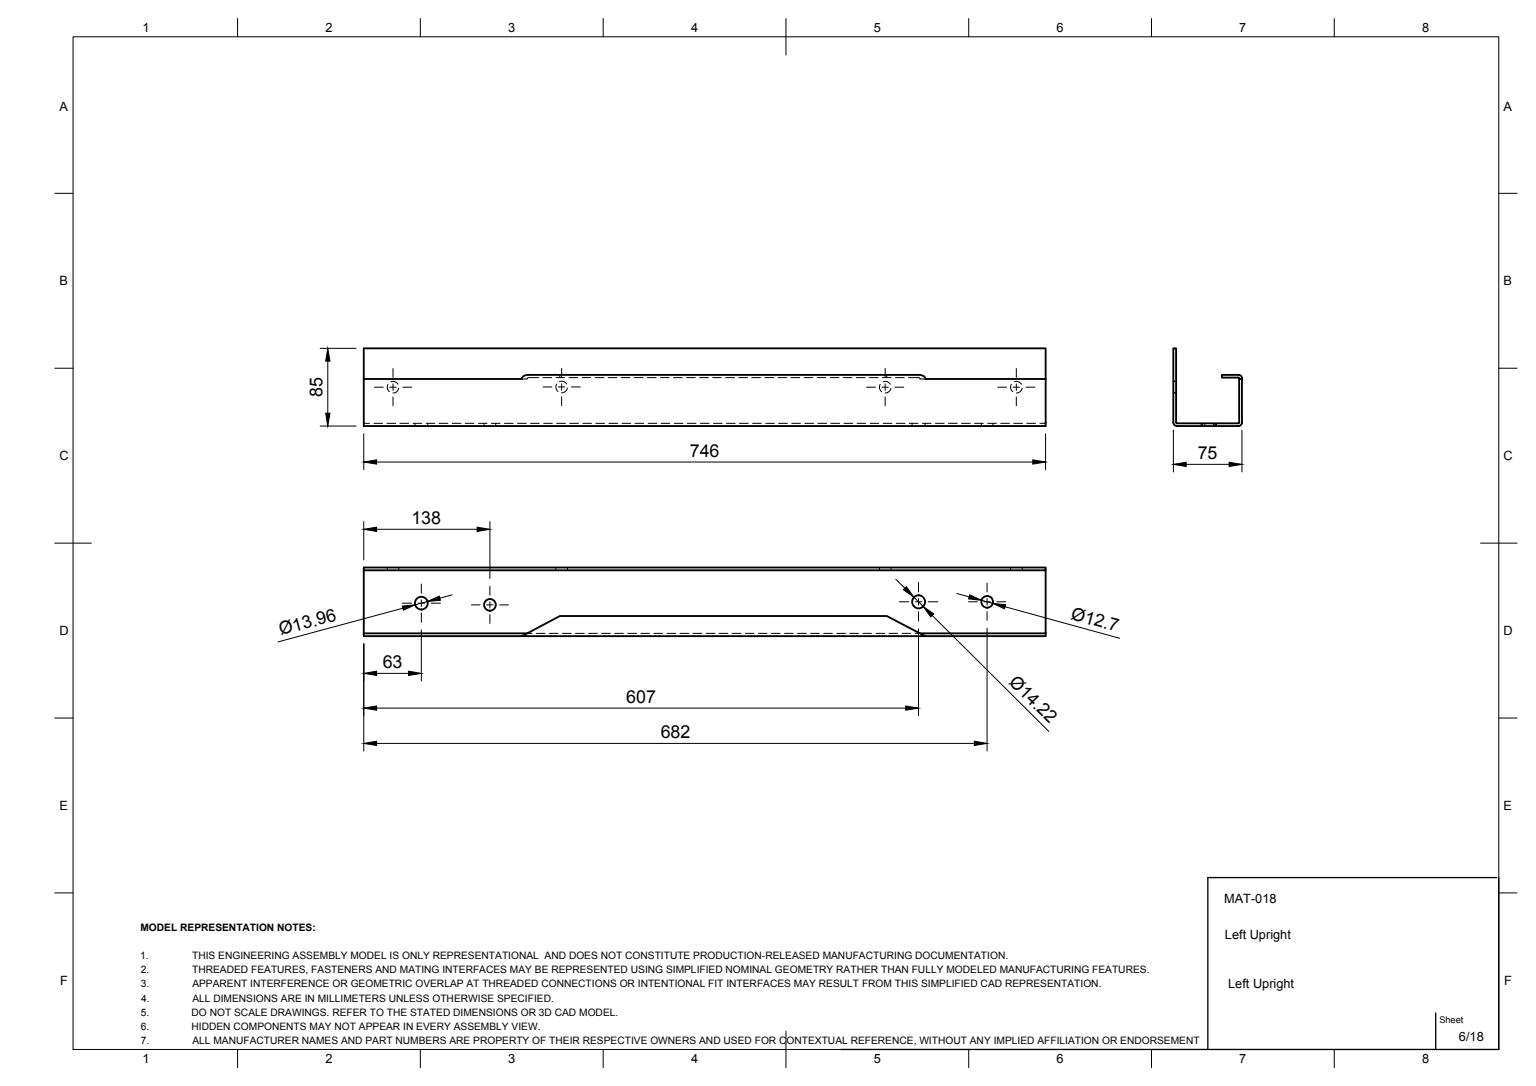
ISO-10303-21;
HEADER;
/* Generated by software containing ST-Developer
 * from STEP Tools, Inc. (www.steptools.com) 
 */

FILE_DESCRIPTION(
/* description */ ('STEP AP214'),
/* implementation_level */ '2;1');

FILE_NAME(
/* name */ 'Left Upright.step',
/* time_stamp */ '2026-11-14T06:16:09-08:00',
/* author */ (''),
/* organization */ (''),
/* preprocessor_version */ 'ST-DEVELOPER v20.2',
/* originating_system */ 'Autodesk Translation Framework v15.17.0.0',
/* authorisation */ '');

FILE_SCHEMA (('AUTOMOTIVE_DESIGN { 1 0 10303 214 3 1 1 }'));
ENDSEC;

DATA;
#10=MECHANICAL_DESIGN_GEOMETRIC_PRESENTATION_REPRESENTATION('',(#350),#18006);
#272=ELLIPSE('',#10126,8.64513309637285,4.00000000000059);
#273=ELLIPSE('',#10127,8.53586336233429,3.99999999999978);
#274=ELLIPSE('',#10140,2.1339658405822,0.999999999999361);
#275=ELLIPSE('',#10141,2.16128327409315,1.00000000000008);
#318=SHAPE_REPRESENTATION_RELATIONSHIP('SRR','None',#18074,#334);
#334=ADVANCED_BREP_SHAPE_REPRESENTATION('',(#366),#17991);
#350=STYLED_ITEM('',(#18171),#366);
#366=MANIFOLD_SOLID_BREP('Body1',#9559);
#433=FACE_BOUND('',#1692,.T.);
#434=FACE_BOUND('',#1693,.T.);
#435=FACE_BOUND('',#1694,.T.);
#436=FACE_BOUND('',#1695,.T.);
#437=FACE_BOUND('',#1698,.T.);
#438=FACE_BOUND('',#1699,.T.);
#439=FACE_BOUND('',#1700,.T.);
#440=FACE_BOUND('',#1701,.T.);
#441=FACE_BOUND('',#1704,.T.);
#442=FACE_BOUND('',#1705,.T.);
#443=FACE_BOUND('',#1706,.T.);
#444=FACE_BOUND('',#1707,.T.);
#445=FACE_BOUND('',#1710,.T.);
#446=FACE_BOUND('',#1711,.T.);
#447=FACE_BOUND('',#1712,.T.);
#448=FACE_BOUND('',#1713,.T.);
#638=PLANE('',#10105);
#639=PLANE('',#10106);
#640=PLANE('',#10109);
#641=PLANE('',#10110);
#642=PLANE('',#10113);
#643=PLANE('',#10114);
#644=PLANE('',#10117);
#645=PLANE('',#10118);
#646=PLANE('',#10121);
#647=PLANE('',#10122);
#648=PLANE('',#10123);
#649=PLANE('',#10124);
#650=PLANE('',#10128);
#651=PLANE('',#10130);
#652=PLANE('',#10132);
#653=PLANE('',#10133);
#654=PLANE('',#10134);
#655=PLANE('',#10136);
#656=PLANE('',#10138);
#657=PLANE('',#10142);
#658=PLANE('',#10143);
#659=PLANE('',#10144);
#660=PLANE('',#10145);
#661=PLANE('',#10146);
#1038=FACE_OUTER_BOUND('',#1668,.T.);
#1039=FACE_OUTER_BOUND('',#1669,.T.);
#1040=FACE_OUTER_BOUND('',#1670,.T.);
#1041=FACE_OUTER_BOUND('',#1671,.T.);
#1042=FACE_OUTER_BOUND('',#1672,.T.);
#1043=FACE_OUTER_BOUND('',#1673,.T.);
#1044=FACE_OUTER_BOUND('',#1674,.T.);
#1045=FACE_OUTER_BOUND('',#1675,.T.);
#1046=FACE_OUTER_BOUND('',#1676,.T.);
#1047=FACE_OUTER_BOUND('',#1677,.T.);
#1048=FACE_OUTER_BOUND('',#1678,.T.);
#1049=FACE_OUTER_BOUND('',#1679,.T.);
#1050=FACE_OUTER_BOUND('',#1680,.T.);
#1051=FACE_OUTER_BOUND('',#1681,.T.);
#1052=FACE_OUTER_BOUND('',#1682,.T.);
#1053=FACE_OUTER_BOUND('',#1683,.T.);
#1054=FACE_OUTER_BOUND('',#1684,.T.);
#1055=FACE_OUTER_BOUND('',#1685,.T.);
#1056=FACE_OUTER_BOUND('',#1686,.T.);
#1057=FACE_OUTER_BOUND('',#1687,.T.);
#1058=FACE_OUTER_BOUND('',#1688,.T.);
#1059=FACE_OUTER_BOUND('',#1689,.T.);
#1060=FACE_OUTER_BOUND('',#1690,.T.);
#1061=FACE_OUTER_BOUND('',#1691,.T.);
#1062=FACE_OUTER_BOUND('',#1696,.T.);
#1063=FACE_OUTER_BOUND('',#1697,.T.);
#1064=FACE_OUTER_BOUND('',#1702,.T.);
#1065=FACE_OUTER_BOUND('',#1703,.T.);
#1066=FACE_OUTER_BOUND('',#1708,.T.);
#1067=FACE_OUTER_BOUND('',#1709,.T.);
#1068=FACE_OUTER_BOUND('',#1714,.T.);
#1069=FACE_OUTER_BOUND('',#1715,.T.);
#1070=FACE_OUTER_BOUND('',#1716,.T.);
#1071=FACE_OUTER_BOUND('',#1717,.T.);
#1072=FACE_OUTER_BOUND('',#1718,.T.);
#1073=FACE_OUTER_BOUND('',#1719,.T.);
#1074=FACE_OUTER_BOUND('',#1720,.T.);
#1075=FACE_OUTER_BOUND('',#1721,.T.);
#1668=EDGE_LOOP('',(#7058,#7059,#7060,#7061));
#1669=EDGE_LOOP('',(#7062,#7063,#7064,#7065));
#1670=EDGE_LOOP('',(#7066,#7067,#7068,#7069));
#1671=EDGE_LOOP('',(#7070,#7071,#7072,#7073));
#1672=EDGE_LOOP('',(#7074,#7075,#7076,#7077));
#1673=EDGE_LOOP('',(#7078,#7079,#7080,#7081));
#1674=EDGE_LOOP('',(#7082,#7083,#7084,#7085));
#1675=EDGE_LOOP('',(#7086,#7087,#7088,#7089));
#1676=EDGE_LOOP('',(#7090,#7091,#7092,#7093));
#1677=EDGE_LOOP('',(#7094,#7095,#7096,#7097));
#1678=EDGE_LOOP('',(#7098,#7099,#7100,#7101));
#1679=EDGE_LOOP('',(#7102,#7103,#7104,#7105));
#1680=EDGE_LOOP('',(#7106,#7107,#7108,#7109));
#1681=EDGE_LOOP('',(#7110,#7111,#7112,#7113));
#1682=EDGE_LOOP('',(#7114,#7115,#7116,#7117));
#1683=EDGE_LOOP('',(#7118,#7119,#7120,#7121));
#1684=EDGE_LOOP('',(#7122,#7123,#7124,#7125));
#1685=EDGE_LOOP('',(#7126,#7127,#7128,#7129));
#1686=EDGE_LOOP('',(#7130,#7131,#7132,#7133));
#1687=EDGE_LOOP('',(#7134,#7135,#7136,#7137));
#1688=EDGE_LOOP('',(#7138,#7139,#7140,#7141));
#1689=EDGE_LOOP('',(#7142,#7143,#7144,#7145,#7146,#7147,#7148,#7149));
#1690=EDGE_LOOP('',(#7150,#7151,#7152,#7153));
#1691=EDGE_LOOP('',(#7154,#7155,#7156,#7157));
#1692=EDGE_LOOP('',(#7158));
#1693=EDGE_LOOP('',(#7159));
#1694=EDGE_LOOP('',(#7160));
#1695=EDGE_LOOP('',(#7161));
#1696=EDGE_LOOP('',(#7162,#7163,#7164,#7165));
#1697=EDGE_LOOP('',(#7166,#7167,#7168,#7169));
#1698=EDGE_LOOP('',(#7170));
#1699=EDGE_LOOP('',(#7171));
#1700=EDGE_LOOP('',(#7172));
#1701=EDGE_LOOP('',(#7173));
#1702=EDGE_LOOP('',(#7174,#7175,#7176,#7177));
#1703=EDGE_LOOP('',(#7178,#7179,#7180,#7181));
#1704=EDGE_LOOP('',(#7182));
#1705=EDGE_LOOP('',(#7183));
#1706=EDGE_LOOP('',(#7184));
#1707=EDGE_LOOP('',(#7185));
#1708=EDGE_LOOP('',(#7186,#7187,#7188,#7189));
#1709=EDGE_LOOP('',(#7190,#7191,#7192,#7193));
#1710=EDGE_LOOP('',(#7194));
#1711=EDGE_LOOP('',(#7195));
#1712=EDGE_LOOP('',(#7196));
#1713=EDGE_LOOP('',(#7197));
#1714=EDGE_LOOP('',(#7198,#7199,#7200,#7201));
#1715=EDGE_LOOP('',(#7202,#7203,#7204,#7205,#7206,#7207,#7208,#7209));
#1716=EDGE_LOOP('',(#7210,#7211,#7212,#7213));
#1717=EDGE_LOOP('',(#7214,#7215,#7216,#7217));
#1718=EDGE_LOOP('',(#7218,#7219,#7220,#7221));
#1719=EDGE_LOOP('',(#7222,#7223,#7224,#7225,#7226,#7227,#7228,#7229));
#1720=EDGE_LOOP('',(#7230,#7231,#7232,#7233,#7234,#7235,#7236,#7237));
#1721=EDGE_LOOP('',(#7238,#7239,#7240,#7241));
#2439=LINE('',#14730,#3163);
#2440=LINE('',#14736,#3164);
#2441=LINE('',#14742,#3165);
#2442=LINE('',#14748,#3166);
#2443=LINE('',#14754,#3167);
#2444=LINE('',#14760,#3168);
#2445=LINE('',#14766,#3169);
#2446=LINE('',#14772,#3170);
#2447=LINE('',#14777,#3171);
#2448=LINE('',#14779,#3172);
#2449=LINE('',#14781,#3173);
#2450=LINE('',#14782,#3174);
#2451=LINE('',#14786,#3175);
#2452=LINE('',#14790,#3176);
#2453=LINE('',#14794,#3177);
#2454=LINE('',#14796,#3178);
#2455=LINE('',#14797,#3179);
#2456=LINE('',#14801,#3180);
#2457=LINE('',#14805,#3181);
#2458=LINE('',#14809,#3182);
#2459=LINE('',#14811,#3183);
#2460=LINE('',#14812,#3184);
#2461=LINE('',#14816,#3185);
#2462=LINE('',#14820,#3186);
#2463=LINE('',#14823,#3187);
#2464=LINE('',#14824,#3188);
#2465=LINE('',#14831,#3189);
#2466=LINE('',#14832,#3190);
#2467=LINE('',#14833,#3191);
#2468=LINE('',#14837,#3192);
#2469=LINE('',#14839,#3193);
#2470=LINE('',#14841,#3194);
#2471=LINE('',#14842,#3195);
#2472=LINE('',#14845,#3196);
#2473=LINE('',#14847,#3197);
#2474=LINE('',#14848,#3198);
#2475=LINE('',#14851,#3199);
#2476=LINE('',#14853,#3200);
#2477=LINE('',#14854,#3201);
#2478=LINE('',#14860,#3202);
#2479=LINE('',#14863,#3203);
#2480=LINE('',#14865,#3204);
#2481=LINE('',#14866,#3205);
#2482=LINE('',#14867,#3206);
#2483=LINE('',#14868,#3207);
#2484=LINE('',#14870,#3208);
#2485=LINE('',#14872,#3209);
#2486=LINE('',#14874,#3210);
#2487=LINE('',#14877,#3211);
#2488=LINE('',#14878,#3212);
#2489=LINE('',#14881,#3213);
#2490=LINE('',#14882,#3214);
#2491=LINE('',#14884,#3215);
#2492=LINE('',#14885,#3216);
#2493=LINE('',#14887,#3217);
#2494=LINE('',#14889,#3218);
#2495=LINE('',#14891,#3219);
#2496=LINE('',#14894,#3220);
#2497=LINE('',#14896,#3221);
#2498=LINE('',#14898,#3222);
#2499=LINE('',#14900,#3223);
#2500=LINE('',#14901,#3224);
#2501=LINE('',#14907,#3225);
#2502=LINE('',#14910,#3226);
#3163=VECTOR('',#11852,7.11098481470124);
#3164=VECTOR('',#11859,6.34999999871023);
#3165=VECTOR('',#11866,6.34999999999997);
#3166=VECTOR('',#11873,6.98053323984749);
#3167=VECTOR('',#11880,6.35);
#3168=VECTOR('',#11887,6.34999999999999);
#3169=VECTOR('',#11894,6.35);
#3170=VECTOR('',#11901,6.35);
#3171=VECTOR('',#11906,1000.);
#3172=VECTOR('',#11907,1000.);
#3173=VECTOR('',#11908,1000.);
#3174=VECTOR('',#11909,1000.);
#3175=VECTOR('',#11912,1000.);
#3176=VECTOR('',#11915,1000.);
#3177=VECTOR('',#11920,1000.);
#3178=VECTOR('',#11921,1000.);
#3179=VECTOR('',#11922,1000.);
#3180=VECTOR('',#11925,1000.);
#3181=VECTOR('',#11928,1000.);
#3182=VECTOR('',#11933,1000.);
#3183=VECTOR('',#11934,1000.);
#3184=VECTOR('',#11935,1000.);
#3185=VECTOR('',#11938,1000.);
#3186=VECTOR('',#11941,1000.);
#3187=VECTOR('',#11946,1000.);
#3188=VECTOR('',#11947,1000.);
#3189=VECTOR('',#11956,1000.);
#3190=VECTOR('',#11957,1000.);
#3191=VECTOR('',#11958,1000.);
#3192=VECTOR('',#11961,1000.);
#3193=VECTOR('',#11962,1000.);
#3194=VECTOR('',#11963,1000.);
#3195=VECTOR('',#11964,1000.);
#3196=VECTOR('',#11967,1000.);
#3197=VECTOR('',#11968,1000.);
#3198=VECTOR('',#11969,1000.);
#3199=VECTOR('',#11972,1000.);
#3200=VECTOR('',#11973,1000.);
#3201=VECTOR('',#11974,1000.);
#3202=VECTOR('',#11981,1000.);
#3203=VECTOR('',#11984,1000.);
#3204=VECTOR('',#11985,1000.);
#3205=VECTOR('',#11986,1000.);
#3206=VECTOR('',#11987,1000.);
#3207=VECTOR('',#11988,1000.);
#3208=VECTOR('',#11991,1000.);
#3209=VECTOR('',#11994,1000.);
#3210=VECTOR('',#11997,1000.);
#3211=VECTOR('',#12000,1000.);
#3212=VECTOR('',#12001,1000.);
#3213=VECTOR('',#12004,1000.);
#3214=VECTOR('',#12005,1000.);
#3215=VECTOR('',#12008,1000.);
#3216=VECTOR('',#12009,1000.);
#3217=VECTOR('',#12012,1000.);
#3218=VECTOR('',#12015,1000.);
#3219=VECTOR('',#12018,1000.);
#3220=VECTOR('',#12021,1000.);
#3221=VECTOR('',#12022,1000.);
#3222=VECTOR('',#12023,1000.);
#3223=VECTOR('',#12024,1000.);
#3224=VECTOR('',#12025,1000.);
#3225=VECTOR('',#12036,1000.);
#3226=VECTOR('',#12041,1000.);
#3690=CIRCLE('',#10082,7.11098481470124);
#3691=CIRCLE('',#10083,7.11098481470124);
#3692=CIRCLE('',#10085,6.34999999871023);
#3693=CIRCLE('',#10086,6.34999999871023);
#3694=CIRCLE('',#10088,6.34999999999997);
#3695=CIRCLE('',#10089,6.34999999999997);
#3696=CIRCLE('',#10091,6.98053323984749);
#3697=CIRCLE('',#10092,6.98053323984749);
#3698=CIRCLE('',#10094,6.35);
#3699=CIRCLE('',#10095,6.35);
#3700=CIRCLE('',#10097,6.34999999999999);
#3701=CIRCLE('',#10098,6.34999999999999);
#3702=CIRCLE('',#10100,6.35);
#3703=CIRCLE('',#10101,6.35);
#3704=CIRCLE('',#10103,6.35);
#3705=CIRCLE('',#10104,6.35);
#3706=CIRCLE('',#10107,4.);
#3707=CIRCLE('',#10108,1.);
#3708=CIRCLE('',#10111,4.);
#3709=CIRCLE('',#10112,1.);
#3710=CIRCLE('',#10115,4.);
#3711=CIRCLE('',#10116,1.);
#3712=CIRCLE('',#10119,4.);
#3713=CIRCLE('',#10120,1.);
#4275=VERTEX_POINT('',#14727);
#4276=VERTEX_POINT('',#14729);
#4277=VERTEX_POINT('',#14733);
#4278=VERTEX_POINT('',#14735);
#4279=VERTEX_POINT('',#14739);
#4280=VERTEX_POINT('',#14741);
#4281=VERTEX_POINT('',#14745);
#4282=VERTEX_POINT('',#14747);
#4283=VERTEX_POINT('',#14751);
#4284=VERTEX_POINT('',#14753);
#4285=VERTEX_POINT('',#14757);
#4286=VERTEX_POINT('',#14759);
#4287=VERTEX_POINT('',#14763);
#4288=VERTEX_POINT('',#14765);
#4289=VERTEX_POINT('',#14769);
#4290=VERTEX_POINT('',#14771);
#4291=VERTEX_POINT('',#14775);
#4292=VERTEX_POINT('',#14776);
#4293=VERTEX_POINT('',#14778);
#4294=VERTEX_POINT('',#14780);
#4295=VERTEX_POINT('',#14784);
#4296=VERTEX_POINT('',#14785);
#4297=VERTEX_POINT('',#14787);
#4298=VERTEX_POINT('',#14789);
#4299=VERTEX_POINT('',#14793);
#4300=VERTEX_POINT('',#14795);
#4301=VERTEX_POINT('',#14799);
#4302=VERTEX_POINT('',#14800);
#4303=VERTEX_POINT('',#14802);
#4304=VERTEX_POINT('',#14804);
#4305=VERTEX_POINT('',#14808);
#4306=VERTEX_POINT('',#14810);
#4307=VERTEX_POINT('',#14814);
#4308=VERTEX_POINT('',#14815);
#4309=VERTEX_POINT('',#14817);
#4310=VERTEX_POINT('',#14819);
#4311=VERTEX_POINT('',#14829);
#4312=VERTEX_POINT('',#14830);
#4313=VERTEX_POINT('',#14835);
#4314=VERTEX_POINT('',#14836);
#4315=VERTEX_POINT('',#14838);
#4316=VERTEX_POINT('',#14840);
#4317=VERTEX_POINT('',#14844);
#4318=VERTEX_POINT('',#14846);
#4319=VERTEX_POINT('',#14850);
#4320=VERTEX_POINT('',#14852);
#4321=VERTEX_POINT('',#14856);
#4322=VERTEX_POINT('',#14858);
#4323=VERTEX_POINT('',#14862);
#4324=VERTEX_POINT('',#14864);
#4325=VERTEX_POINT('',#14876);
#4326=VERTEX_POINT('',#14880);
#4327=VERTEX_POINT('',#14893);
#4328=VERTEX_POINT('',#14895);
#4329=VERTEX_POINT('',#14897);
#4330=VERTEX_POINT('',#14899);
#5277=EDGE_CURVE('',#4275,#4275,#3690,.T.);
#5278=EDGE_CURVE('',#4275,#4276,#2439,.T.);
#5279=EDGE_CURVE('',#4276,#4276,#3691,.T.);
#5280=EDGE_CURVE('',#4277,#4277,#3692,.T.);
#5281=EDGE_CURVE('',#4277,#4278,#2440,.T.);
#5282=EDGE_CURVE('',#4278,#4278,#3693,.T.);
#5283=EDGE_CURVE('',#4279,#4279,#3694,.T.);
#5284=EDGE_CURVE('',#4279,#4280,#2441,.T.);
#5285=EDGE_CURVE('',#4280,#4280,#3695,.T.);
#5286=EDGE_CURVE('',#4281,#4281,#3696,.T.);
#5287=EDGE_CURVE('',#4281,#4282,#2442,.T.);
#5288=EDGE_CURVE('',#4282,#4282,#3697,.T.);
#5289=EDGE_CURVE('',#4283,#4283,#3698,.T.);
#5290=EDGE_CURVE('',#4283,#4284,#2443,.T.);
#5291=EDGE_CURVE('',#4284,#4284,#3699,.T.);
#5292=EDGE_CURVE('',#4285,#4285,#3700,.T.);
#5293=EDGE_CURVE('',#4285,#4286,#2444,.T.);
#5294=EDGE_CURVE('',#4286,#4286,#3701,.T.);
#5295=EDGE_CURVE('',#4287,#4287,#3702,.T.);
#5296=EDGE_CURVE('',#4287,#4288,#2445,.T.);
#5297=EDGE_CURVE('',#4288,#4288,#3703,.T.);
#5298=EDGE_CURVE('',#4289,#4289,#3704,.T.);
#5299=EDGE_CURVE('',#4289,#4290,#2446,.T.);
#5300=EDGE_CURVE('',#4290,#4290,#3705,.T.);
#5301=EDGE_CURVE('',#4291,#4292,#2447,.T.);
#5302=EDGE_CURVE('',#4293,#4291,#2448,.T.);
#5303=EDGE_CURVE('',#4293,#4294,#2449,.T.);
#5304=EDGE_CURVE('',#4292,#4294,#2450,.T.);
#5305=EDGE_CURVE('',#4295,#4296,#2451,.T.);
#5306=EDGE_CURVE('',#4296,#4297,#3706,.T.);
#5307=EDGE_CURVE('',#4297,#4298,#2452,.T.);
#5308=EDGE_CURVE('',#4295,#4298,#3707,.T.);
#5309=EDGE_CURVE('',#4299,#4295,#2453,.T.);
#5310=EDGE_CURVE('',#4299,#4300,#2454,.T.);
#5311=EDGE_CURVE('',#4300,#4296,#2455,.T.);
#5312=EDGE_CURVE('',#4301,#4302,#2456,.T.);
#5313=EDGE_CURVE('',#4303,#4302,#3708,.T.);
#5314=EDGE_CURVE('',#4303,#4304,#2457,.T.);
#5315=EDGE_CURVE('',#4304,#4301,#3709,.T.);
#5316=EDGE_CURVE('',#4301,#4305,#2458,.T.);
#5317=EDGE_CURVE('',#4306,#4305,#2459,.T.);
#5318=EDGE_CURVE('',#4302,#4306,#2460,.T.);
#5319=EDGE_CURVE('',#4307,#4308,#2461,.T.);
#5320=EDGE_CURVE('',#4308,#4309,#3710,.T.);
#5321=EDGE_CURVE('',#4309,#4310,#2462,.T.);
#5322=EDGE_CURVE('',#4307,#4310,#3711,.T.);
#5323=EDGE_CURVE('',#4298,#4307,#2463,.T.);
#5324=EDGE_CURVE('',#4297,#4308,#2464,.T.);
#5325=EDGE_CURVE('',#4306,#4291,#3712,.T.);
#5326=EDGE_CURVE('',#4305,#4293,#3713,.T.);
#5327=EDGE_CURVE('',#4311,#4312,#2465,.T.);
#5328=EDGE_CURVE('',#4310,#4312,#2466,.T.);
#5329=EDGE_CURVE('',#4309,#4311,#2467,.T.);
#5330=EDGE_CURVE('',#4313,#4314,#2468,.T.);
#5331=EDGE_CURVE('',#4315,#4313,#2469,.T.);
#5332=EDGE_CURVE('',#4315,#4316,#2470,.T.);
#5333=EDGE_CURVE('',#4314,#4316,#2471,.T.);
#5334=EDGE_CURVE('',#4316,#4317,#2472,.T.);
#5335=EDGE_CURVE('',#4315,#4318,#2473,.T.);
#5336=EDGE_CURVE('',#4318,#4317,#2474,.T.);
#5337=EDGE_CURVE('',#4319,#4317,#2475,.T.);
#5338=EDGE_CURVE('',#4318,#4320,#2476,.T.);
#5339=EDGE_CURVE('',#4320,#4319,#2477,.T.);
#5340=EDGE_CURVE('',#4321,#4319,#272,.T.);
#5341=EDGE_CURVE('',#4320,#4322,#273,.T.);
#5342=EDGE_CURVE('',#4322,#4321,#2478,.T.);
#5343=EDGE_CURVE('',#4323,#4321,#2479,.T.);
#5344=EDGE_CURVE('',#4322,#4324,#2480,.T.);
#5345=EDGE_CURVE('',#4324,#4311,#2481,.T.);
#5346=EDGE_CURVE('',#4309,#4291,#2482,.T.);
#5347=EDGE_CURVE('',#4323,#4292,#2483,.T.);
#5348=EDGE_CURVE('',#4308,#4306,#2484,.T.);
#5349=EDGE_CURVE('',#4297,#4302,#2485,.T.);
#5350=EDGE_CURVE('',#4296,#4303,#2486,.T.);
#5351=EDGE_CURVE('',#4325,#4303,#2487,.T.);
#5352=EDGE_CURVE('',#4300,#4325,#2488,.T.);
#5353=EDGE_CURVE('',#4326,#4325,#2489,.T.);
#5354=EDGE_CURVE('',#4299,#4326,#2490,.T.);
#5355=EDGE_CURVE('',#4326,#4304,#2491,.T.);
#5356=EDGE_CURVE('',#4295,#4304,#2492,.T.);
#5357=EDGE_CURVE('',#4298,#4301,#2493,.T.);
#5358=EDGE_CURVE('',#4307,#4305,#2494,.T.);
#5359=EDGE_CURVE('',#4310,#4293,#2495,.T.);
#5360=EDGE_CURVE('',#4327,#4294,#2496,.T.);
#5361=EDGE_CURVE('',#4328,#4312,#2497,.T.);
#5362=EDGE_CURVE('',#4329,#4328,#2498,.T.);
#5363=EDGE_CURVE('',#4329,#4330,#2499,.T.);
#5364=EDGE_CURVE('',#4327,#4330,#2500,.T.);
#5365=EDGE_CURVE('',#4313,#4329,#274,.T.);
#5366=EDGE_CURVE('',#4330,#4314,#275,.T.);
#5367=EDGE_CURVE('',#4328,#4324,#2501,.T.);
#5368=EDGE_CURVE('',#4323,#4327,#2502,.T.);
#7058=ORIENTED_EDGE('',*,*,#5277,.F.);
#7059=ORIENTED_EDGE('',*,*,#5278,.T.);
#7060=ORIENTED_EDGE('',*,*,#5279,.T.);
#7061=ORIENTED_EDGE('',*,*,#5278,.F.);
#7062=ORIENTED_EDGE('',*,*,#5280,.T.);
#7063=ORIENTED_EDGE('',*,*,#5281,.T.);
#7064=ORIENTED_EDGE('',*,*,#5282,.F.);
#7065=ORIENTED_EDGE('',*,*,#5281,.F.);
#7066=ORIENTED_EDGE('',*,*,#5283,.T.);
#7067=ORIENTED_EDGE('',*,*,#5284,.T.);
#7068=ORIENTED_EDGE('',*,*,#5285,.F.);
#7069=ORIENTED_EDGE('',*,*,#5284,.F.);
#7070=ORIENTED_EDGE('',*,*,#5286,.T.);
#7071=ORIENTED_EDGE('',*,*,#5287,.T.);
#7072=ORIENTED_EDGE('',*,*,#5288,.F.);
#7073=ORIENTED_EDGE('',*,*,#5287,.F.);
#7074=ORIENTED_EDGE('',*,*,#5289,.T.);
#7075=ORIENTED_EDGE('',*,*,#5290,.T.);
#7076=ORIENTED_EDGE('',*,*,#5291,.F.);
#7077=ORIENTED_EDGE('',*,*,#5290,.F.);
#7078=ORIENTED_EDGE('',*,*,#5292,.T.);
#7079=ORIENTED_EDGE('',*,*,#5293,.T.);
#7080=ORIENTED_EDGE('',*,*,#5294,.F.);
#7081=ORIENTED_EDGE('',*,*,#5293,.F.);
#7082=ORIENTED_EDGE('',*,*,#5295,.T.);
#7083=ORIENTED_EDGE('',*,*,#5296,.T.);
#7084=ORIENTED_EDGE('',*,*,#5297,.F.);
#7085=ORIENTED_EDGE('',*,*,#5296,.F.);
#7086=ORIENTED_EDGE('',*,*,#5298,.T.);
#7087=ORIENTED_EDGE('',*,*,#5299,.T.);
#7088=ORIENTED_EDGE('',*,*,#5300,.F.);
#7089=ORIENTED_EDGE('',*,*,#5299,.F.);
#7090=ORIENTED_EDGE('',*,*,#5301,.F.);
#7091=ORIENTED_EDGE('',*,*,#5302,.F.);
#7092=ORIENTED_EDGE('',*,*,#5303,.T.);
#7093=ORIENTED_EDGE('',*,*,#5304,.F.);
#7094=ORIENTED_EDGE('',*,*,#5305,.T.);
#7095=ORIENTED_EDGE('',*,*,#5306,.T.);
#7096=ORIENTED_EDGE('',*,*,#5307,.T.);
#7097=ORIENTED_EDGE('',*,*,#5308,.F.);
#7098=ORIENTED_EDGE('',*,*,#5309,.F.);
#7099=ORIENTED_EDGE('',*,*,#5310,.T.);
#7100=ORIENTED_EDGE('',*,*,#5311,.T.);
#7101=ORIENTED_EDGE('',*,*,#5305,.F.);
#7102=ORIENTED_EDGE('',*,*,#5312,.T.);
#7103=ORIENTED_EDGE('',*,*,#5313,.F.);
#7104=ORIENTED_EDGE('',*,*,#5314,.T.);
#7105=ORIENTED_EDGE('',*,*,#5315,.T.);
#7106=ORIENTED_EDGE('',*,*,#5316,.T.);
#7107=ORIENTED_EDGE('',*,*,#5317,.F.);
#7108=ORIENTED_EDGE('',*,*,#5318,.F.);
#7109=ORIENTED_EDGE('',*,*,#5312,.F.);
#7110=ORIENTED_EDGE('',*,*,#5319,.T.);
#7111=ORIENTED_EDGE('',*,*,#5320,.T.);
#7112=ORIENTED_EDGE('',*,*,#5321,.T.);
#7113=ORIENTED_EDGE('',*,*,#5322,.F.);
#7114=ORIENTED_EDGE('',*,*,#5323,.F.);
#7115=ORIENTED_EDGE('',*,*,#5307,.F.);
#7116=ORIENTED_EDGE('',*,*,#5324,.T.);
#7117=ORIENTED_EDGE('',*,*,#5319,.F.);
#7118=ORIENTED_EDGE('',*,*,#5302,.T.);
#7119=ORIENTED_EDGE('',*,*,#5325,.F.);
#7120=ORIENTED_EDGE('',*,*,#5317,.T.);
#7121=ORIENTED_EDGE('',*,*,#5326,.T.);
#7122=ORIENTED_EDGE('',*,*,#5327,.T.);
#7123=ORIENTED_EDGE('',*,*,#5328,.F.);
#7124=ORIENTED_EDGE('',*,*,#5321,.F.);
#7125=ORIENTED_EDGE('',*,*,#5329,.T.);
#7126=ORIENTED_EDGE('',*,*,#5330,.F.);
#7127=ORIENTED_EDGE('',*,*,#5331,.F.);
#7128=ORIENTED_EDGE('',*,*,#5332,.T.);
#7129=ORIENTED_EDGE('',*,*,#5333,.F.);
#7130=ORIENTED_EDGE('',*,*,#5334,.F.);
#7131=ORIENTED_EDGE('',*,*,#5332,.F.);
#7132=ORIENTED_EDGE('',*,*,#5335,.T.);
#7133=ORIENTED_EDGE('',*,*,#5336,.T.);
#7134=ORIENTED_EDGE('',*,*,#5337,.T.);
#7135=ORIENTED_EDGE('',*,*,#5336,.F.);
#7136=ORIENTED_EDGE('',*,*,#5338,.T.);
#7137=ORIENTED_EDGE('',*,*,#5339,.T.);
#7138=ORIENTED_EDGE('',*,*,#5340,.T.);
#7139=ORIENTED_EDGE('',*,*,#5339,.F.);
#7140=ORIENTED_EDGE('',*,*,#5341,.T.);
#7141=ORIENTED_EDGE('',*,*,#5342,.T.);
#7142=ORIENTED_EDGE('',*,*,#5343,.T.);
#7143=ORIENTED_EDGE('',*,*,#5342,.F.);
#7144=ORIENTED_EDGE('',*,*,#5344,.T.);
#7145=ORIENTED_EDGE('',*,*,#5345,.T.);
#7146=ORIENTED_EDGE('',*,*,#5329,.F.);
#7147=ORIENTED_EDGE('',*,*,#5346,.T.);
#7148=ORIENTED_EDGE('',*,*,#5301,.T.);
#7149=ORIENTED_EDGE('',*,*,#5347,.F.);
#7150=ORIENTED_EDGE('',*,*,#5325,.T.);
#7151=ORIENTED_EDGE('',*,*,#5346,.F.);
#7152=ORIENTED_EDGE('',*,*,#5320,.F.);
#7153=ORIENTED_EDGE('',*,*,#5348,.T.);
#7154=ORIENTED_EDGE('',*,*,#5318,.T.);
#7155=ORIENTED_EDGE('',*,*,#5348,.F.);
#7156=ORIENTED_EDGE('',*,*,#5324,.F.);
#7157=ORIENTED_EDGE('',*,*,#5349,.T.);
#7158=ORIENTED_EDGE('',*,*,#5279,.F.);
#7159=ORIENTED_EDGE('',*,*,#5282,.T.);
#7160=ORIENTED_EDGE('',*,*,#5285,.T.);
#7161=ORIENTED_EDGE('',*,*,#5288,.T.);
#7162=ORIENTED_EDGE('',*,*,#5313,.T.);
#7163=ORIENTED_EDGE('',*,*,#5349,.F.);
#7164=ORIENTED_EDGE('',*,*,#5306,.F.);
#7165=ORIENTED_EDGE('',*,*,#5350,.T.);
#7166=ORIENTED_EDGE('',*,*,#5351,.T.);
#7167=ORIENTED_EDGE('',*,*,#5350,.F.);
#7168=ORIENTED_EDGE('',*,*,#5311,.F.);
#7169=ORIENTED_EDGE('',*,*,#5352,.T.);
#7170=ORIENTED_EDGE('',*,*,#5291,.T.);
#7171=ORIENTED_EDGE('',*,*,#5294,.T.);
#7172=ORIENTED_EDGE('',*,*,#5297,.T.);
#7173=ORIENTED_EDGE('',*,*,#5300,.T.);
#7174=ORIENTED_EDGE('',*,*,#5353,.T.);
#7175=ORIENTED_EDGE('',*,*,#5352,.F.);
#7176=ORIENTED_EDGE('',*,*,#5310,.F.);
#7177=ORIENTED_EDGE('',*,*,#5354,.T.);
#7178=ORIENTED_EDGE('',*,*,#5355,.F.);
#7179=ORIENTED_EDGE('',*,*,#5354,.F.);
#7180=ORIENTED_EDGE('',*,*,#5309,.T.);
#7181=ORIENTED_EDGE('',*,*,#5356,.T.);
#7182=ORIENTED_EDGE('',*,*,#5289,.F.);
#7183=ORIENTED_EDGE('',*,*,#5292,.F.);
#7184=ORIENTED_EDGE('',*,*,#5295,.F.);
#7185=ORIENTED_EDGE('',*,*,#5298,.F.);
#7186=ORIENTED_EDGE('',*,*,#5315,.F.);
#7187=ORIENTED_EDGE('',*,*,#5356,.F.);
#7188=ORIENTED_EDGE('',*,*,#5308,.T.);
#7189=ORIENTED_EDGE('',*,*,#5357,.T.);
#7190=ORIENTED_EDGE('',*,*,#5316,.F.);
#7191=ORIENTED_EDGE('',*,*,#5357,.F.);
#7192=ORIENTED_EDGE('',*,*,#5323,.T.);
#7193=ORIENTED_EDGE('',*,*,#5358,.T.);
#7194=ORIENTED_EDGE('',*,*,#5277,.T.);
#7195=ORIENTED_EDGE('',*,*,#5280,.F.);
#7196=ORIENTED_EDGE('',*,*,#5283,.F.);
#7197=ORIENTED_EDGE('',*,*,#5286,.F.);
#7198=ORIENTED_EDGE('',*,*,#5326,.F.);
#7199=ORIENTED_EDGE('',*,*,#5358,.F.);
#7200=ORIENTED_EDGE('',*,*,#5322,.T.);
#7201=ORIENTED_EDGE('',*,*,#5359,.T.);
#7202=ORIENTED_EDGE('',*,*,#5360,.T.);
#7203=ORIENTED_EDGE('',*,*,#5303,.F.);
#7204=ORIENTED_EDGE('',*,*,#5359,.F.);
#7205=ORIENTED_EDGE('',*,*,#5328,.T.);
#7206=ORIENTED_EDGE('',*,*,#5361,.F.);
#7207=ORIENTED_EDGE('',*,*,#5362,.F.);
#7208=ORIENTED_EDGE('',*,*,#5363,.T.);
#7209=ORIENTED_EDGE('',*,*,#5364,.F.);
#7210=ORIENTED_EDGE('',*,*,#5363,.F.);
#7211=ORIENTED_EDGE('',*,*,#5365,.F.);
#7212=ORIENTED_EDGE('',*,*,#5330,.T.);
#7213=ORIENTED_EDGE('',*,*,#5366,.F.);
#7214=ORIENTED_EDGE('',*,*,#5351,.F.);
#7215=ORIENTED_EDGE('',*,*,#5353,.F.);
#7216=ORIENTED_EDGE('',*,*,#5355,.T.);
#7217=ORIENTED_EDGE('',*,*,#5314,.F.);
#7218=ORIENTED_EDGE('',*,*,#5345,.F.);
#7219=ORIENTED_EDGE('',*,*,#5367,.F.);
#7220=ORIENTED_EDGE('',*,*,#5361,.T.);
#7221=ORIENTED_EDGE('',*,*,#5327,.F.);
#7222=ORIENTED_EDGE('',*,*,#5341,.F.);
#7223=ORIENTED_EDGE('',*,*,#5338,.F.);
#7224=ORIENTED_EDGE('',*,*,#5335,.F.);
#7225=ORIENTED_EDGE('',*,*,#5331,.T.);
#7226=ORIENTED_EDGE('',*,*,#5365,.T.);
#7227=ORIENTED_EDGE('',*,*,#5362,.T.);
#7228=ORIENTED_EDGE('',*,*,#5367,.T.);
#7229=ORIENTED_EDGE('',*,*,#5344,.F.);
#7230=ORIENTED_EDGE('',*,*,#5340,.F.);
#7231=ORIENTED_EDGE('',*,*,#5343,.F.);
#7232=ORIENTED_EDGE('',*,*,#5368,.T.);
#7233=ORIENTED_EDGE('',*,*,#5364,.T.);
#7234=ORIENTED_EDGE('',*,*,#5366,.T.);
#7235=ORIENTED_EDGE('',*,*,#5333,.T.);
#7236=ORIENTED_EDGE('',*,*,#5334,.T.);
#7237=ORIENTED_EDGE('',*,*,#5337,.F.);
#7238=ORIENTED_EDGE('',*,*,#5368,.F.);
#7239=ORIENTED_EDGE('',*,*,#5347,.T.);
#7240=ORIENTED_EDGE('',*,*,#5304,.T.);
#7241=ORIENTED_EDGE('',*,*,#5360,.F.);
#8869=CYLINDRICAL_SURFACE('',#10081,7.11098481470124);
#8870=CYLINDRICAL_SURFACE('',#10084,6.34999999871023);
#8871=CYLINDRICAL_SURFACE('',#10087,6.34999999999997);
#8872=CYLINDRICAL_SURFACE('',#10090,6.98053323984749);
#8873=CYLINDRICAL_SURFACE('',#10093,6.35);
#8874=CYLINDRICAL_SURFACE('',#10096,6.34999999999999);
#8875=CYLINDRICAL_SURFACE('',#10099,6.35);
#8876=CYLINDRICAL_SURFACE('',#10102,6.35);
#8877=CYLINDRICAL_SURFACE('',#10125,4.);
#8878=CYLINDRICAL_SURFACE('',#10129,4.);
#8879=CYLINDRICAL_SURFACE('',#10131,4.);
#8880=CYLINDRICAL_SURFACE('',#10135,1.);
#8881=CYLINDRICAL_SURFACE('',#10137,1.);
#8882=CYLINDRICAL_SURFACE('',#10139,1.);
#9177=ADVANCED_FACE('',(#1038),#8869,.F.);
#9178=ADVANCED_FACE('',(#1039),#8870,.F.);
#9179=ADVANCED_FACE('',(#1040),#8871,.F.);
#9180=ADVANCED_FACE('',(#1041),#8872,.F.);
#9181=ADVANCED_FACE('',(#1042),#8873,.F.);
#9182=ADVANCED_FACE('',(#1043),#8874,.F.);
#9183=ADVANCED_FACE('',(#1044),#8875,.F.);
#9184=ADVANCED_FACE('',(#1045),#8876,.F.);
#9185=ADVANCED_FACE('',(#1046),#638,.T.);
#9186=ADVANCED_FACE('',(#1047),#639,.T.);
#9187=ADVANCED_FACE('',(#1048),#640,.T.);
#9188=ADVANCED_FACE('',(#1049),#641,.T.);
#9189=ADVANCED_FACE('',(#1050),#642,.T.);
#9190=ADVANCED_FACE('',(#1051),#643,.T.);
#9191=ADVANCED_FACE('',(#1052),#644,.T.);
#9192=ADVANCED_FACE('',(#1053),#645,.T.);
#9193=ADVANCED_FACE('',(#1054),#646,.T.);
#9194=ADVANCED_FACE('',(#1055),#647,.F.);
#9195=ADVANCED_FACE('',(#1056),#648,.T.);
#9196=ADVANCED_FACE('',(#1057),#649,.T.);
#9197=ADVANCED_FACE('',(#1058),#8877,.T.);
#9198=ADVANCED_FACE('',(#1059),#650,.T.);
#9199=ADVANCED_FACE('',(#1060),#8878,.T.);
#9200=ADVANCED_FACE('',(#1061,#433,#434,#435,#436),#651,.T.);
#9201=ADVANCED_FACE('',(#1062),#8879,.T.);
#9202=ADVANCED_FACE('',(#1063,#437,#438,#439,#440),#652,.T.);
#9203=ADVANCED_FACE('',(#1064),#653,.T.);
#9204=ADVANCED_FACE('',(#1065,#441,#442,#443,#444),#654,.F.);
#9205=ADVANCED_FACE('',(#1066),#8880,.F.);
#9206=ADVANCED_FACE('',(#1067,#445,#446,#447,#448),#655,.F.);
#9207=ADVANCED_FACE('',(#1068),#8881,.F.);
#9208=ADVANCED_FACE('',(#1069),#656,.F.);
#9209=ADVANCED_FACE('',(#1070),#8882,.F.);
#9210=ADVANCED_FACE('',(#1071),#657,.F.);
#9211=ADVANCED_FACE('',(#1072),#658,.F.);
#9212=ADVANCED_FACE('',(#1073),#659,.F.);
#9213=ADVANCED_FACE('',(#1074),#660,.F.);
#9214=ADVANCED_FACE('',(#1075),#661,.T.);
#9559=CLOSED_SHELL('',(#9177,#9178,#9179,#9180,#9181,#9182,#9183,#9184,
#9185,#9186,#9187,#9188,#9189,#9190,#9191,#9192,#9193,#9194,#9195,#9196,
#9197,#9198,#9199,#9200,#9201,#9202,#9203,#9204,#9205,#9206,#9207,#9208,
#9209,#9210,#9211,#9212,#9213,#9214));
#10080=AXIS2_PLACEMENT_3D('',#14725,#11846,#11847);
#10081=AXIS2_PLACEMENT_3D('',#14726,#11848,#11849);
#10082=AXIS2_PLACEMENT_3D('',#14728,#11850,#11851);
#10083=AXIS2_PLACEMENT_3D('',#14731,#11853,#11854);
#10084=AXIS2_PLACEMENT_3D('',#14732,#11855,#11856);
#10085=AXIS2_PLACEMENT_3D('',#14734,#11857,#11858);
#10086=AXIS2_PLACEMENT_3D('',#14737,#11860,#11861);
#10087=AXIS2_PLACEMENT_3D('',#14738,#11862,#11863);
#10088=AXIS2_PLACEMENT_3D('',#14740,#11864,#11865);
#10089=AXIS2_PLACEMENT_3D('',#14743,#11867,#11868);
#10090=AXIS2_PLACEMENT_3D('',#14744,#11869,#11870);
#10091=AXIS2_PLACEMENT_3D('',#14746,#11871,#11872);
#10092=AXIS2_PLACEMENT_3D('',#14749,#11874,#11875);
#10093=AXIS2_PLACEMENT_3D('',#14750,#11876,#11877);
#10094=AXIS2_PLACEMENT_3D('',#14752,#11878,#11879);
#10095=AXIS2_PLACEMENT_3D('',#14755,#11881,#11882);
#10096=AXIS2_PLACEMENT_3D('',#14756,#11883,#11884);
#10097=AXIS2_PLACEMENT_3D('',#14758,#11885,#11886);
#10098=AXIS2_PLACEMENT_3D('',#14761,#11888,#11889);
#10099=AXIS2_PLACEMENT_3D('',#14762,#11890,#11891);
#10100=AXIS2_PLACEMENT_3D('',#14764,#11892,#11893);
#10101=AXIS2_PLACEMENT_3D('',#14767,#11895,#11896);
#10102=AXIS2_PLACEMENT_3D('',#14768,#11897,#11898);
#10103=AXIS2_PLACEMENT_3D('',#14770,#11899,#11900);
#10104=AXIS2_PLACEMENT_3D('',#14773,#11902,#11903);
#10105=AXIS2_PLACEMENT_3D('',#14774,#11904,#11905);
#10106=AXIS2_PLACEMENT_3D('',#14783,#11910,#11911);
#10107=AXIS2_PLACEMENT_3D('',#14788,#11913,#11914);
#10108=AXIS2_PLACEMENT_3D('',#14791,#11916,#11917);
#10109=AXIS2_PLACEMENT_3D('',#14792,#11918,#11919);
#10110=AXIS2_PLACEMENT_3D('',#14798,#11923,#11924);
#10111=AXIS2_PLACEMENT_3D('',#14803,#11926,#11927);
#10112=AXIS2_PLACEMENT_3D('',#14806,#11929,#11930);
#10113=AXIS2_PLACEMENT_3D('',#14807,#11931,#11932);
#10114=AXIS2_PLACEMENT_3D('',#14813,#11936,#11937);
#10115=AXIS2_PLACEMENT_3D('',#14818,#11939,#11940);
#10116=AXIS2_PLACEMENT_3D('',#14821,#11942,#11943);
#10117=AXIS2_PLACEMENT_3D('',#14822,#11944,#11945);
#10118=AXIS2_PLACEMENT_3D('',#14825,#11948,#11949);
#10119=AXIS2_PLACEMENT_3D('',#14826,#11950,#11951);
#10120=AXIS2_PLACEMENT_3D('',#14827,#11952,#11953);
#10121=AXIS2_PLACEMENT_3D('',#14828,#11954,#11955);
#10122=AXIS2_PLACEMENT_3D('',#14834,#11959,#11960);
#10123=AXIS2_PLACEMENT_3D('',#14843,#11965,#11966);
#10124=AXIS2_PLACEMENT_3D('',#14849,#11970,#11971);
#10125=AXIS2_PLACEMENT_3D('',#14855,#11975,#11976);
#10126=AXIS2_PLACEMENT_3D('',#14857,#11977,#11978);
#10127=AXIS2_PLACEMENT_3D('',#14859,#11979,#11980);
#10128=AXIS2_PLACEMENT_3D('',#14861,#11982,#11983);
#10129=AXIS2_PLACEMENT_3D('',#14869,#11989,#11990);
#10130=AXIS2_PLACEMENT_3D('',#14871,#11992,#11993);
#10131=AXIS2_PLACEMENT_3D('',#14873,#11995,#11996);
#10132=AXIS2_PLACEMENT_3D('',#14875,#11998,#11999);
#10133=AXIS2_PLACEMENT_3D('',#14879,#12002,#12003);
#10134=AXIS2_PLACEMENT_3D('',#14883,#12006,#12007);
#10135=AXIS2_PLACEMENT_3D('',#14886,#12010,#12011);
#10136=AXIS2_PLACEMENT_3D('',#14888,#12013,#12014);
#10137=AXIS2_PLACEMENT_3D('',#14890,#12016,#12017);
#10138=AXIS2_PLACEMENT_3D('',#14892,#12019,#12020);
#10139=AXIS2_PLACEMENT_3D('',#14902,#12026,#12027);
#10140=AXIS2_PLACEMENT_3D('',#14903,#12028,#12029);
#10141=AXIS2_PLACEMENT_3D('',#14904,#12030,#12031);
#10142=AXIS2_PLACEMENT_3D('',#14905,#12032,#12033);
#10143=AXIS2_PLACEMENT_3D('',#14906,#12034,#12035);
#10144=AXIS2_PLACEMENT_3D('',#14908,#12037,#12038);
#10145=AXIS2_PLACEMENT_3D('',#14909,#12039,#12040);
#10146=AXIS2_PLACEMENT_3D('',#14911,#12042,#12043);
#11846=DIRECTION('axis',(0.,0.,1.));
#11847=DIRECTION('refdir',(1.,0.,0.));
#11848=DIRECTION('center_axis',(-1.,0.,0.));
#11849=DIRECTION('ref_axis',(0.,0.,1.));
#11850=DIRECTION('center_axis',(-1.,0.,0.));
#11851=DIRECTION('ref_axis',(0.,0.,1.));
#11852=DIRECTION('',(-1.,0.,0.));
#11853=DIRECTION('center_axis',(-1.,0.,0.));
#11854=DIRECTION('ref_axis',(0.,0.,1.));
#11855=DIRECTION('center_axis',(-1.,0.,0.));
#11856=DIRECTION('ref_axis',(0.,0.,-1.));
#11857=DIRECTION('center_axis',(1.,0.,0.));
#11858=DIRECTION('ref_axis',(0.,0.,-1.));
#11859=DIRECTION('',(-1.,0.,0.));
#11860=DIRECTION('center_axis',(1.,0.,0.));
#11861=DIRECTION('ref_axis',(0.,0.,-1.));
#11862=DIRECTION('center_axis',(-1.,0.,0.));
#11863=DIRECTION('ref_axis',(0.,0.,-1.));
#11864=DIRECTION('center_axis',(1.,0.,0.));
#11865=DIRECTION('ref_axis',(0.,0.,-1.));
#11866=DIRECTION('',(-1.,0.,0.));
#11867=DIRECTION('center_axis',(1.,0.,0.));
#11868=DIRECTION('ref_axis',(0.,0.,-1.));
#11869=DIRECTION('center_axis',(-1.,0.,0.));
#11870=DIRECTION('ref_axis',(0.,0.,-1.));
#11871=DIRECTION('center_axis',(1.,0.,0.));
#11872=DIRECTION('ref_axis',(0.,0.,-1.));
#11873=DIRECTION('',(-1.,0.,0.));
#11874=DIRECTION('center_axis',(1.,0.,0.));
#11875=DIRECTION('ref_axis',(0.,0.,-1.));
#11876=DIRECTION('center_axis',(1.22464679914735E-16,-1.,0.));
#11877=DIRECTION('ref_axis',(1.,1.22464679914735E-16,0.));
#11878=DIRECTION('center_axis',(-1.22464679914735E-16,1.,0.));
#11879=DIRECTION('ref_axis',(1.,1.22464679914735E-16,0.));
#11880=DIRECTION('',(1.22464679914735E-16,-1.,0.));
#11881=DIRECTION('center_axis',(-1.22464679914735E-16,1.,0.));
#11882=DIRECTION('ref_axis',(1.,1.22464679914735E-16,0.));
#11883=DIRECTION('center_axis',(1.22464679914735E-16,-1.,0.));
#11884=DIRECTION('ref_axis',(1.,1.22464679914735E-16,0.));
#11885=DIRECTION('center_axis',(-1.22464679914735E-16,1.,0.));
#11886=DIRECTION('ref_axis',(1.,1.22464679914735E-16,0.));
#11887=DIRECTION('',(1.22464679914735E-16,-1.,0.));
#11888=DIRECTION('center_axis',(-1.22464679914735E-16,1.,0.));
#11889=DIRECTION('ref_axis',(-1.,-1.22464679914735E-16,0.));
#11890=DIRECTION('center_axis',(1.22464679914735E-16,-1.,0.));
#11891=DIRECTION('ref_axis',(1.,1.22464679914735E-16,0.));
#11892=DIRECTION('center_axis',(-1.22464679914735E-16,1.,0.));
#11893=DIRECTION('ref_axis',(1.,1.22464679914735E-16,0.));
#11894=DIRECTION('',(1.22464679914735E-16,-1.,0.));
#11895=DIRECTION('center_axis',(-1.22464679914735E-16,1.,0.));
#11896=DIRECTION('ref_axis',(1.,1.22464679914735E-16,0.));
#11897=DIRECTION('center_axis',(1.22464679914735E-16,-1.,0.));
#11898=DIRECTION('ref_axis',(1.,1.22464679914735E-16,0.));
#11899=DIRECTION('center_axis',(-1.22464679914735E-16,1.,0.));
#11900=DIRECTION('ref_axis',(1.,1.22464679914735E-16,0.));
#11901=DIRECTION('',(1.22464679914735E-16,-1.,0.));
#11902=DIRECTION('center_axis',(-1.22464679914735E-16,1.,0.));
#11903=DIRECTION('ref_axis',(1.,1.22464679914735E-16,0.));
#11904=DIRECTION('center_axis',(0.,0.,1.));
#11905=DIRECTION('ref_axis',(-1.,0.,0.));
#11906=DIRECTION('',(1.,0.,0.));
#11907=DIRECTION('',(0.,1.,0.));
#11908=DIRECTION('',(1.,0.,0.));
#11909=DIRECTION('',(0.,-1.,0.));
#11910=DIRECTION('center_axis',(0.,0.,-1.));
#11911=DIRECTION('ref_axis',(1.,0.,0.));
#11912=DIRECTION('',(0.,-1.,0.));
#11913=DIRECTION('center_axis',(0.,0.,-1.));
#11914=DIRECTION('ref_axis',(1.,0.,0.));
#11915=DIRECTION('',(1.,0.,0.));
#11916=DIRECTION('center_axis',(0.,0.,-1.));
#11917=DIRECTION('ref_axis',(1.,0.,0.));
#11918=DIRECTION('center_axis',(0.,0.,-1.));
#11919=DIRECTION('ref_axis',(1.,0.,0.));
#11920=DIRECTION('',(-1.,-1.22464679914735E-16,0.));
#11921=DIRECTION('',(1.22464679914735E-16,-1.,0.));
#11922=DIRECTION('',(-1.,-1.22464679914735E-16,0.));
#11923=DIRECTION('center_axis',(0.,0.,1.));
#11924=DIRECTION('ref_axis',(-1.,0.,0.));
#11925=DIRECTION('',(-1.,0.,0.));
#11926=DIRECTION('center_axis',(0.,0.,-1.));
#11927=DIRECTION('ref_axis',(1.,0.,0.));
#11928=DIRECTION('',(0.,1.,0.));
#11929=DIRECTION('center_axis',(0.,0.,-1.));
#11930=DIRECTION('ref_axis',(1.,0.,0.));
#11931=DIRECTION('center_axis',(0.,0.,1.));
#11932=DIRECTION('ref_axis',(-1.,0.,0.));
#11933=DIRECTION('',(0.,1.,0.));
#11934=DIRECTION('',(1.,0.,0.));
#11935=DIRECTION('',(0.,1.,0.));
#11936=DIRECTION('center_axis',(0.,0.,-1.));
#11937=DIRECTION('ref_axis',(1.,0.,0.));
#11938=DIRECTION('',(-1.,0.,0.));
#11939=DIRECTION('center_axis',(0.,0.,-1.));
#11940=DIRECTION('ref_axis',(1.,0.,0.));
#11941=DIRECTION('',(0.,-1.,0.));
#11942=DIRECTION('center_axis',(0.,0.,-1.));
#11943=DIRECTION('ref_axis',(1.,0.,0.));
#11944=DIRECTION('center_axis',(0.,0.,-1.));
#11945=DIRECTION('ref_axis',(1.,0.,0.));
#11946=DIRECTION('',(0.,1.,0.));
#11947=DIRECTION('',(0.,1.,0.));
#11948=DIRECTION('center_axis',(0.,0.,1.));
#11949=DIRECTION('ref_axis',(-1.,0.,0.));
#11950=DIRECTION('center_axis',(0.,0.,-1.));
#11951=DIRECTION('ref_axis',(1.,0.,0.));
#11952=DIRECTION('center_axis',(0.,0.,-1.));
#11953=DIRECTION('ref_axis',(1.,0.,0.));
#11954=DIRECTION('center_axis',(0.,0.,-1.));
#11955=DIRECTION('ref_axis',(1.,0.,0.));
#11956=DIRECTION('',(0.,-1.,0.));
#11957=DIRECTION('',(1.,0.,0.));
#11958=DIRECTION('',(1.,0.,0.));
#11959=DIRECTION('center_axis',(1.,-3.65204942310907E-16,0.));
#11960=DIRECTION('ref_axis',(3.65204942310907E-16,1.,0.));
#11961=DIRECTION('',(0.,0.,1.));
#11962=DIRECTION('',(1.71139076064604E-16,0.468611062549393,-0.883404591371547));
#11963=DIRECTION('',(0.,0.,1.));
#11964=DIRECTION('',(-1.68975972140531E-16,-0.462688076101332,-0.886521147087675));
#11965=DIRECTION('center_axis',(0.,-1.,0.));
#11966=DIRECTION('ref_axis',(0.,0.,1.));
#11967=DIRECTION('',(1.,0.,0.));
#11968=DIRECTION('',(1.,0.,0.));
#11969=DIRECTION('',(0.,0.,1.));
#11970=DIRECTION('center_axis',(1.,-3.65204942310907E-16,0.));
#11971=DIRECTION('ref_axis',(3.65204942310907E-16,1.,0.));
#11972=DIRECTION('',(0.,-0.462688076101332,-0.886521147087675));
#11973=DIRECTION('',(0.,0.468611062549393,-0.883404591371547));
#11974=DIRECTION('',(0.,0.,1.));
#11975=DIRECTION('center_axis',(0.,0.,1.));
#11976=DIRECTION('ref_axis',(-1.,0.,0.));
#11977=DIRECTION('center_axis',(9.04452389970748E-15,0.886521147087677,
-0.462688076101329));
#11978=DIRECTION('ref_axis',(8.69090002824443E-14,0.462688076101329,0.886521147087677));
#11979=DIRECTION('center_axis',(1.79450933059916E-14,0.88340459137155,0.468611062549386));
#11980=DIRECTION('ref_axis',(1.21092278199327E-14,-0.468611062549386,0.88340459137155));
#11981=DIRECTION('',(0.,0.,1.));
#11982=DIRECTION('center_axis',(0.,1.,0.));
#11983=DIRECTION('ref_axis',(0.,0.,-1.));
#11984=DIRECTION('',(1.,0.,0.));
#11985=DIRECTION('',(-1.,0.,0.));
#11986=DIRECTION('',(0.,0.,-1.));
#11987=DIRECTION('',(0.,0.,1.));
#11988=DIRECTION('',(0.,0.,1.));
#11989=DIRECTION('center_axis',(0.,0.,1.));
#11990=DIRECTION('ref_axis',(-1.,0.,0.));
#11991=DIRECTION('',(0.,0.,1.));
#11992=DIRECTION('center_axis',(-1.,0.,0.));
#11993=DIRECTION('ref_axis',(0.,0.,-1.));
#11994=DIRECTION('',(0.,0.,1.));
#11995=DIRECTION('center_axis',(0.,0.,1.));
#11996=DIRECTION('ref_axis',(-1.,0.,0.));
#11997=DIRECTION('',(0.,0.,1.));
#11998=DIRECTION('center_axis',(1.22464679914735E-16,-1.,0.));
#11999=DIRECTION('ref_axis',(1.,1.22464679914735E-16,0.));
#12000=DIRECTION('',(-1.,-1.22464679914735E-16,0.));
#12001=DIRECTION('',(0.,0.,1.));
#12002=DIRECTION('center_axis',(1.,1.22464679914735E-16,0.));
#12003=DIRECTION('ref_axis',(-1.22464679914735E-16,1.,0.));
#12004=DIRECTION('',(1.22464679914735E-16,-1.,0.));
#12005=DIRECTION('',(0.,0.,1.));
#12006=DIRECTION('center_axis',(1.22464679914735E-16,-1.,0.));
#12007=DIRECTION('ref_axis',(1.,1.22464679914735E-16,0.));
#12008=DIRECTION('',(-1.,-1.22464679914735E-16,0.));
#12009=DIRECTION('',(0.,0.,1.));
#12010=DIRECTION('center_axis',(0.,0.,1.));
#12011=DIRECTION('ref_axis',(-1.,0.,0.));
#12012=DIRECTION('',(0.,0.,1.));
#12013=DIRECTION('center_axis',(-1.,0.,0.));
#12014=DIRECTION('ref_axis',(0.,0.,-1.));
#12015=DIRECTION('',(0.,0.,1.));
#12016=DIRECTION('center_axis',(0.,0.,1.));
#12017=DIRECTION('ref_axis',(-1.,0.,0.));
#12018=DIRECTION('',(0.,0.,1.));
#12019=DIRECTION('center_axis',(0.,1.,0.));
#12020=DIRECTION('ref_axis',(0.,0.,-1.));
#12021=DIRECTION('',(0.,0.,1.));
#12022=DIRECTION('',(0.,0.,-1.));
#12023=DIRECTION('',(-1.,0.,0.));
#12024=DIRECTION('',(0.,0.,1.));
#12025=DIRECTION('',(1.,0.,0.));
#12026=DIRECTION('center_axis',(0.,0.,1.));
#12027=DIRECTION('ref_axis',(-1.,0.,0.));
#12028=DIRECTION('center_axis',(-1.88700981155792E-14,0.883404591371546,
0.468611062549393));
#12029=DIRECTION('ref_axis',(3.43055792298147E-13,-0.468611062549393,0.883404591371546));
#12030=DIRECTION('center_axis',(2.77796091205298E-14,0.886521147087676,
-0.462688076101331));
#12031=DIRECTION('ref_axis',(6.62185632336808E-14,0.462688076101331,0.886521147087676));
#12032=DIRECTION('center_axis',(0.,0.,-1.));
#12033=DIRECTION('ref_axis',(1.,0.,0.));
#12034=DIRECTION('center_axis',(-1.,0.,0.));
#12035=DIRECTION('ref_axis',(0.,0.,-1.));
#12036=DIRECTION('',(0.,0.468611062549393,-0.883404591371547));
#12037=DIRECTION('center_axis',(0.,0.883404591371547,0.468611062549393));
#12038=DIRECTION('ref_axis',(0.,0.468611062549393,-0.883404591371547));
#12039=DIRECTION('center_axis',(0.,0.886521147087676,-0.462688076101332));
#12040=DIRECTION('ref_axis',(0.,-0.462688076101332,-0.886521147087676));
#12041=DIRECTION('',(0.,-0.462688076101332,-0.886521147087675));
#12042=DIRECTION('center_axis',(1.,0.,0.));
#12043=DIRECTION('ref_axis',(0.,0.,1.));
#14725=CARTESIAN_POINT('',(0.,0.,0.));
#14726=CARTESIAN_POINT('Origin',(-81.58,34.5,-138.999999999993));
#14727=CARTESIAN_POINT('',(-82.,34.5,-146.110984814694));
#14728=CARTESIAN_POINT('Origin',(-82.,34.5,-138.999999999993));
#14729=CARTESIAN_POINT('',(-85.,34.5,-146.110984814694));
#14730=CARTESIAN_POINT('',(-81.58,34.5,-146.110984814694));
#14731=CARTESIAN_POINT('Origin',(-85.,34.5,-138.999999999993));
#14732=CARTESIAN_POINT('Origin',(-81.58,34.5,-63.9999999999928));
#14733=CARTESIAN_POINT('',(-82.,34.5,-57.6500000012826));
#14734=CARTESIAN_POINT('Origin',(-82.,34.5,-63.9999999999928));
#14735=CARTESIAN_POINT('',(-85.,34.5,-57.6500000012826));
#14736=CARTESIAN_POINT('',(-81.58,34.5,-57.6500000012826));
#14737=CARTESIAN_POINT('Origin',(-85.,34.5,-63.9999999999928));
#14738=CARTESIAN_POINT('Origin',(-81.58,37.8359855953527,-608.));
#14739=CARTESIAN_POINT('',(-82.,37.8359855953527,-601.65));
#14740=CARTESIAN_POINT('Origin',(-82.,37.8359855953527,-608.));
#14741=CARTESIAN_POINT('',(-85.,37.8359855953527,-601.65));
#14742=CARTESIAN_POINT('',(-81.58,37.8359855953527,-601.65));
#14743=CARTESIAN_POINT('Origin',(-85.,37.8359855953527,-608.));
#14744=CARTESIAN_POINT('Origin',(-81.58,35.9826602646012,-683.));
#14745=CARTESIAN_POINT('',(-82.,35.9826602646012,-676.019466760152));
#14746=CARTESIAN_POINT('Origin',(-82.,35.9826602646012,-683.));
#14747=CARTESIAN_POINT('',(-85.,35.9826602646012,-676.019466760152));
#14748=CARTESIAN_POINT('',(-81.58,35.9826602646012,-676.019466760152));
#14749=CARTESIAN_POINT('Origin',(-85.,35.9826602646012,-683.));
#14750=CARTESIAN_POINT('Origin',(-42.5,1.49999999999999,-32.0000000000144));
#14751=CARTESIAN_POINT('',(-48.85,-6.10622663543836E-15,-32.0000000000144));
#14752=CARTESIAN_POINT('Origin',(-42.5,-5.20417042793042E-15,-32.0000000000144));
#14753=CARTESIAN_POINT('',(-48.85,-3.00000000000001,-32.0000000000144));
#14754=CARTESIAN_POINT('',(-48.85,1.49999999999999,-32.0000000000144));
#14755=CARTESIAN_POINT('Origin',(-42.5,-3.00000000000001,-32.0000000000144));
#14756=CARTESIAN_POINT('Origin',(-42.5000000000001,1.49999999999999,-713.999999999986));
#14757=CARTESIAN_POINT('',(-48.8500000000001,-6.10622663543836E-15,-713.999999999986));
#14758=CARTESIAN_POINT('Origin',(-42.5000000000001,-5.20417042793042E-15,
-713.999999999986));
#14759=CARTESIAN_POINT('',(-48.8500000000001,-3.00000000000001,-713.999999999986));
#14760=CARTESIAN_POINT('',(-48.8500000000001,1.49999999999999,-713.999999999986));
#14761=CARTESIAN_POINT('Origin',(-42.5000000000001,-3.00000000000001,-713.999999999986));
#14762=CARTESIAN_POINT('Origin',(-42.2900000000001,1.49999999999999,-529.5));
#14763=CARTESIAN_POINT('',(-48.6400000000001,-6.10622663543836E-15,-529.5));
#14764=CARTESIAN_POINT('Origin',(-42.2900000000001,-5.20417042793042E-15,
-529.5));
#14765=CARTESIAN_POINT('',(-48.6400000000001,-3.00000000000001,-529.5));
#14766=CARTESIAN_POINT('',(-48.6400000000001,1.49999999999999,-529.5));
#14767=CARTESIAN_POINT('Origin',(-42.2900000000001,-3.00000000000001,-529.5));
#14768=CARTESIAN_POINT('Origin',(-42.5,1.49999999999999,-175.500000000014));
#14769=CARTESIAN_POINT('',(-48.85,-6.10622663543836E-15,-175.500000000014));
#14770=CARTESIAN_POINT('Origin',(-42.5,-5.20417042793042E-15,-175.500000000014));
#14771=CARTESIAN_POINT('',(-48.85,-3.00000000000001,-175.500000000014));
#14772=CARTESIAN_POINT('',(-48.85,1.49999999999999,-175.500000000014));
#14773=CARTESIAN_POINT('Origin',(-42.5,-3.00000000000001,-175.500000000014));
#14774=CARTESIAN_POINT('Origin',(-85.,68.,0.));
#14775=CARTESIAN_POINT('',(-81.,72.,0.));
#14776=CARTESIAN_POINT('',(-33.5,72.,0.));
#14777=CARTESIAN_POINT('',(-82.,72.,0.));
#14778=CARTESIAN_POINT('',(-81.,69.,0.));
#14779=CARTESIAN_POINT('',(-81.,69.,0.));
#14780=CARTESIAN_POINT('',(-33.5,69.,0.));
#14781=CARTESIAN_POINT('',(-82.,69.,0.));
#14782=CARTESIAN_POINT('',(-33.5,68.,0.));
#14783=CARTESIAN_POINT('Origin',(-81.,-9.91963907309357E-15,-746.));
#14784=CARTESIAN_POINT('',(-81.,-9.91963907309357E-15,-746.));
#14785=CARTESIAN_POINT('',(-81.,-3.00000000000001,-746.));
#14786=CARTESIAN_POINT('',(-81.,-9.91963907309357E-15,-746.));
#14787=CARTESIAN_POINT('',(-85.,0.99999999999999,-746.));
#14788=CARTESIAN_POINT('Origin',(-81.,0.99999999999999,-746.));
#14789=CARTESIAN_POINT('',(-82.,0.99999999999999,-746.));
#14790=CARTESIAN_POINT('',(-85.,0.99999999999999,-746.));
#14791=CARTESIAN_POINT('Origin',(-81.,0.99999999999999,-746.));
#14792=CARTESIAN_POINT('Origin',(-85.,0.99999999999999,-746.));
#14793=CARTESIAN_POINT('',(0.,0.,-746.));
#14794=CARTESIAN_POINT('',(0.,0.,-746.));
#14795=CARTESIAN_POINT('',(3.67394039744206E-16,-3.,-746.));
#14796=CARTESIAN_POINT('',(0.,0.,-746.));
#14797=CARTESIAN_POINT('',(3.67394039744206E-16,-3.,-746.));
#14798=CARTESIAN_POINT('Origin',(-82.,0.99999999999999,0.));
#14799=CARTESIAN_POINT('',(-82.,0.99999999999999,0.));
#14800=CARTESIAN_POINT('',(-85.,0.99999999999999,0.));
#14801=CARTESIAN_POINT('',(-82.,0.99999999999999,0.));
#14802=CARTESIAN_POINT('',(-81.,-3.00000000000001,0.));
#14803=CARTESIAN_POINT('Origin',(-81.,0.99999999999999,0.));
#14804=CARTESIAN_POINT('',(-81.,-9.91963907309357E-15,0.));
#14805=CARTESIAN_POINT('',(-81.,-3.00000000000001,0.));
#14806=CARTESIAN_POINT('Origin',(-81.,0.99999999999999,0.));
#14807=CARTESIAN_POINT('Origin',(-81.,-3.00000000000001,0.));
#14808=CARTESIAN_POINT('',(-82.,68.,0.));
#14809=CARTESIAN_POINT('',(-82.,-1.00421037530083E-14,0.));
#14810=CARTESIAN_POINT('',(-85.,68.,0.));
#14811=CARTESIAN_POINT('',(-85.,68.,0.));
#14812=CARTESIAN_POINT('',(-85.,-1.00421037530083E-14,0.));
#14813=CARTESIAN_POINT('Origin',(-82.,68.,-746.));
#14814=CARTESIAN_POINT('',(-82.,68.,-746.));
#14815=CARTESIAN_POINT('',(-85.,68.,-746.));
#14816=CARTESIAN_POINT('',(-82.,68.,-746.));
#14817=CARTESIAN_POINT('',(-81.,72.,-746.));
#14818=CARTESIAN_POINT('Origin',(-81.,68.,-746.));
#14819=CARTESIAN_POINT('',(-81.,69.,-746.));
#14820=CARTESIAN_POINT('',(-81.,72.,-746.));
#14821=CARTESIAN_POINT('Origin',(-81.,68.,-746.));
#14822=CARTESIAN_POINT('Origin',(-81.,72.,-746.));
#14823=CARTESIAN_POINT('',(-82.,-1.00421037530083E-14,-746.));
#14824=CARTESIAN_POINT('',(-85.,-1.00421037530083E-14,-746.));
#14825=CARTESIAN_POINT('Origin',(-81.,69.,0.));
#14826=CARTESIAN_POINT('Origin',(-81.,68.,0.));
#14827=CARTESIAN_POINT('Origin',(-81.,68.,0.));
#14828=CARTESIAN_POINT('Origin',(-29.,68.,-746.));
#14829=CARTESIAN_POINT('',(-33.5,72.,-746.));
#14830=CARTESIAN_POINT('',(-33.5,69.,-746.));
#14831=CARTESIAN_POINT('',(-33.5,50.,-746.));
#14832=CARTESIAN_POINT('',(-82.,69.,-746.));
#14833=CARTESIAN_POINT('',(-82.,72.,-746.));
#14834=CARTESIAN_POINT('Origin',(-32.,69.,-746.));
#14835=CARTESIAN_POINT('',(-32.,68.,-565.447580013871));
#14836=CARTESIAN_POINT('',(-32.,68.,-139.329431198143));
#14837=CARTESIAN_POINT('',(-32.,68.,-746.));
#14838=CARTESIAN_POINT('',(-32.,50.,-531.514786028642));
#14839=CARTESIAN_POINT('',(-32.,142.963452937836,-706.765324733926));
#14840=CARTESIAN_POINT('',(-32.,50.,-173.817851090086));
#14841=CARTESIAN_POINT('',(-32.,50.,-746.));
#14842=CARTESIAN_POINT('',(-32.0000000000001,-180.631730474111,-615.713626701011));
#14843=CARTESIAN_POINT('Origin',(-29.,50.,-746.));
#14844=CARTESIAN_POINT('',(-29.,50.,-173.817851090086));
#14845=CARTESIAN_POINT('',(-33.5,50.,-173.817851090086));
#14846=CARTESIAN_POINT('',(-29.,50.,-531.514786028642));
#14847=CARTESIAN_POINT('',(-33.5,50.,-531.514786028642));
#14848=CARTESIAN_POINT('',(-29.,50.,-746.));
#14849=CARTESIAN_POINT('Origin',(-29.,69.,-746.));
#14850=CARTESIAN_POINT('',(-29.,68.,-139.329431198143));
#14851=CARTESIAN_POINT('',(-29.,50.,-173.817851090086));
#14852=CARTESIAN_POINT('',(-29.,68.,-565.447580013871));
#14853=CARTESIAN_POINT('',(-29.,72.6655742581807,-574.242911687517));
#14854=CARTESIAN_POINT('',(-29.,68.,-746.));
#14855=CARTESIAN_POINT('Origin',(-33.,68.,-746.));
#14856=CARTESIAN_POINT('',(-33.,72.,-131.665337888822));
#14857=CARTESIAN_POINT('Origin',(-33.0000000000006,67.9999999999993,-139.329431198144));
#14858=CARTESIAN_POINT('',(-33.,72.,-572.988200899477));
#14859=CARTESIAN_POINT('Origin',(-32.9999999999998,68.0000000000002,-565.447580013871));
#14860=CARTESIAN_POINT('',(-33.,72.,-746.));
#14861=CARTESIAN_POINT('Origin',(-82.,72.,-746.));
#14862=CARTESIAN_POINT('',(-33.5,72.,-131.665337888822));
#14863=CARTESIAN_POINT('',(-82.,72.,-131.665337888822));
#14864=CARTESIAN_POINT('',(-33.5,72.,-572.988200899477));
#14865=CARTESIAN_POINT('',(-82.,72.,-572.988200899477));
#14866=CARTESIAN_POINT('',(-33.5,72.,-746.));
#14867=CARTESIAN_POINT('',(-81.,72.,-746.));
#14868=CARTESIAN_POINT('',(-33.5,72.,-746.));
#14869=CARTESIAN_POINT('Origin',(-81.,68.,-746.));
#14870=CARTESIAN_POINT('',(-85.,68.,-746.));
#14871=CARTESIAN_POINT('Origin',(-85.,-1.00421037530083E-14,-746.));
#14872=CARTESIAN_POINT('',(-85.,0.99999999999999,-746.));
#14873=CARTESIAN_POINT('Origin',(-81.,0.99999999999999,-746.));
#14874=CARTESIAN_POINT('',(-81.,-3.00000000000001,-746.));
#14875=CARTESIAN_POINT('Origin',(3.67394039744206E-16,-3.,-746.));
#14876=CARTESIAN_POINT('',(3.67394039744206E-16,-3.,0.));
#14877=CARTESIAN_POINT('',(3.67394039744206E-16,-3.,0.));
#14878=CARTESIAN_POINT('',(3.67394039744206E-16,-3.,-746.));
#14879=CARTESIAN_POINT('Origin',(0.,0.,-746.));
#14880=CARTESIAN_POINT('',(0.,0.,0.));
#14881=CARTESIAN_POINT('',(0.,0.,0.));
#14882=CARTESIAN_POINT('',(0.,0.,-746.));
#14883=CARTESIAN_POINT('Origin',(0.,0.,-746.));
#14884=CARTESIAN_POINT('',(0.,0.,0.));
#14885=CARTESIAN_POINT('',(-81.,-9.91963907309357E-15,-746.));
#14886=CARTESIAN_POINT('Origin',(-81.,0.99999999999999,-746.));
#14887=CARTESIAN_POINT('',(-82.,0.99999999999999,-746.));
#14888=CARTESIAN_POINT('Origin',(-82.,-1.00421037530083E-14,-746.));
#14889=CARTESIAN_POINT('',(-82.,68.,-746.));
#14890=CARTESIAN_POINT('Origin',(-81.,68.,-746.));
#14891=CARTESIAN_POINT('',(-81.,69.,-746.));
#14892=CARTESIAN_POINT('Origin',(-82.,69.,-746.));
#14893=CARTESIAN_POINT('',(-33.5,69.,-137.413407870812));
#14894=CARTESIAN_POINT('',(-33.5,69.,-746.));
#14895=CARTESIAN_POINT('',(-33.5,69.,-567.332735235272));
#14896=CARTESIAN_POINT('',(-33.5,69.,-746.));
#14897=CARTESIAN_POINT('',(-33.,69.,-567.332735235272));
#14898=CARTESIAN_POINT('',(-82.,69.,-567.332735235272));
#14899=CARTESIAN_POINT('',(-33.,69.,-137.413407870813));
#14900=CARTESIAN_POINT('',(-33.,69.,-746.));
#14901=CARTESIAN_POINT('',(-82.,69.,-137.413407870813));
#14902=CARTESIAN_POINT('Origin',(-33.,68.,-746.));
#14903=CARTESIAN_POINT('Origin',(-32.9999999999994,68.0000000000007,-565.447580013872));
#14904=CARTESIAN_POINT('Origin',(-33.0000000000001,67.9999999999998,-139.329431198143));
#14905=CARTESIAN_POINT('Origin',(-33.,68.,0.));
#14906=CARTESIAN_POINT('Origin',(-33.5,0.,0.));
#14907=CARTESIAN_POINT('',(-33.5,72.6655742581807,-574.242911687517));
#14908=CARTESIAN_POINT('Origin',(-33.5,72.6655742581807,-574.242911687517));
#14909=CARTESIAN_POINT('Origin',(-33.5,50.,-173.817851090086));
#14910=CARTESIAN_POINT('',(-33.5,50.,-173.817851090086));
#14911=CARTESIAN_POINT('Origin',(-33.5,0.,0.));
#17971=UNCERTAINTY_MEASURE_WITH_UNIT(LENGTH_MEASURE(0.01),#18007,
'DISTANCE_ACCURACY_VALUE',
'Maximum model space distance between geometric entities at asserted c
onnectivities');
#17986=UNCERTAINTY_MEASURE_WITH_UNIT(LENGTH_MEASURE(0.01),#18007,
'DISTANCE_ACCURACY_VALUE',
'Maximum model space distance between geometric entities at asserted c
onnectivities');
#17991=(
GEOMETRIC_REPRESENTATION_CONTEXT(3)
GLOBAL_UNCERTAINTY_ASSIGNED_CONTEXT((#17971))
GLOBAL_UNIT_ASSIGNED_CONTEXT((#18007,#18009,#18010))
REPRESENTATION_CONTEXT('','3D')
);
#18006=(
GEOMETRIC_REPRESENTATION_CONTEXT(3)
GLOBAL_UNCERTAINTY_ASSIGNED_CONTEXT((#17986))
GLOBAL_UNIT_ASSIGNED_CONTEXT((#18007,#18009,#18010))
REPRESENTATION_CONTEXT('','3D')
);
#18007=(
LENGTH_UNIT()
NAMED_UNIT(*)
SI_UNIT(.MILLI.,.METRE.)
);
#18009=(
NAMED_UNIT(*)
PLANE_ANGLE_UNIT()
SI_UNIT($,.RADIAN.)
);
#18010=(
NAMED_UNIT(*)
SI_UNIT($,.STERADIAN.)
SOLID_ANGLE_UNIT()
);
#18015=SHAPE_DEFINITION_REPRESENTATION(#18034,#18074);
#18034=PRODUCT_DEFINITION_SHAPE('',$,#18094);
#18074=SHAPE_REPRESENTATION('',(#10080),#17991);
#18089=PRODUCT_DEFINITION_CONTEXT('part definition',#18148,'design');
#18094=PRODUCT_DEFINITION('Left Upright','Left Upright',#18113,#18089);
#18113=PRODUCT_DEFINITION_FORMATION('',$,#18154);
#18148=APPLICATION_CONTEXT(
'Core Data for Automotive Mechanical Design Process');
#18149=PRODUCT_CONTEXT('part definition',#18148,'mechanical');
#18154=PRODUCT('Left Upright','Left Upright',$,(#18149));
#18171=PRESENTATION_STYLE_ASSIGNMENT((#18175));
#18175=SURFACE_STYLE_USAGE(.BOTH.,#18179);
#18179=SURFACE_SIDE_STYLE('',(#18183));
#18183=SURFACE_STYLE_FILL_AREA(#18187);
#18187=FILL_AREA_STYLE('Opaque(61,176,222)',(#18191));
#18191=FILL_AREA_STYLE_COLOUR('Opaque(61,176,222)',#18195);
#18195=COLOUR_RGB('Opaque(61,176,222)',0.23921568627451,0.690196078431373,
0.870588235294118);
ENDSEC;
END-ISO-10303-21;
